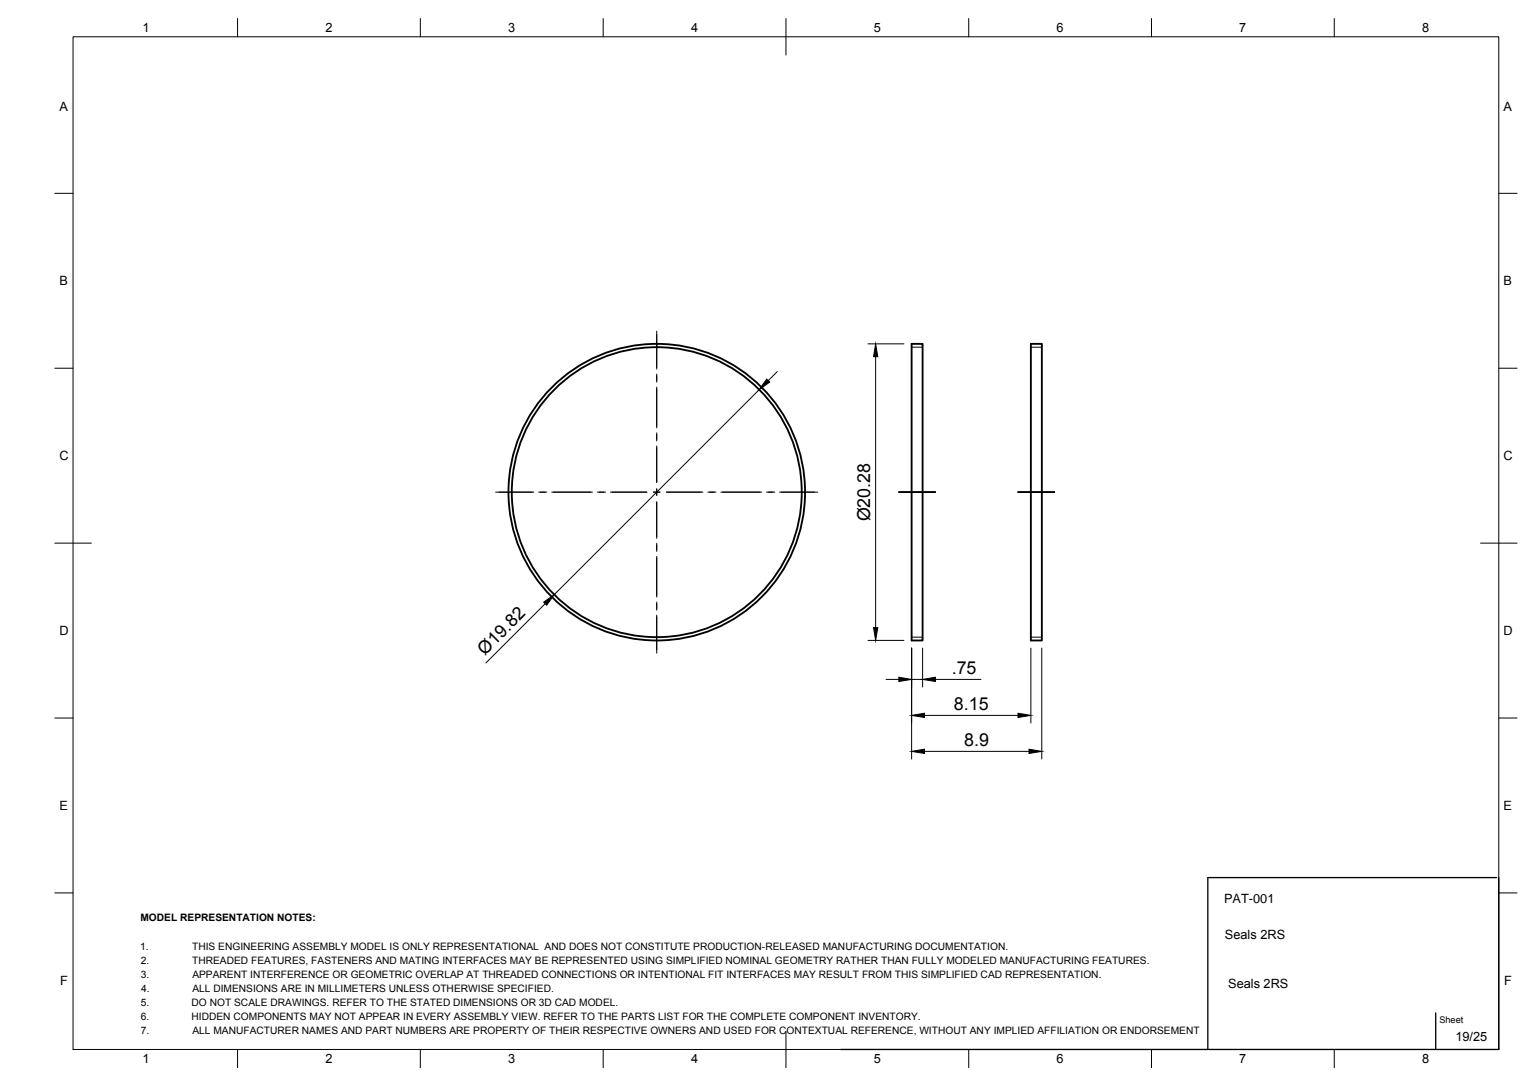
ISO-10303-21;
HEADER;
/* Generated by software containing ST-Developer
 * from STEP Tools, Inc. (www.steptools.com) 
 */

FILE_DESCRIPTION(
/* description */ ('PAT-001'),
/* implementation_level */ '2;1');

FILE_NAME(
/* name */ 'Seals 2RS.step',
/* time_stamp */ '2026-10-29T17:07:15-07:00',
/* author */ (''),
/* organization */ (''),
/* preprocessor_version */ 'ST-DEVELOPER v20.2',
/* originating_system */ 'Autodesk Translation Framework v15.17.0.0',
/* authorisation */ '');

FILE_SCHEMA (('AUTOMOTIVE_DESIGN { 1 0 10303 214 3 1 1 }'));
ENDSEC;

DATA;
#10=MECHANICAL_DESIGN_GEOMETRIC_PRESENTATION_REPRESENTATION('',(#389,#390),#9622);
#332=SHAPE_REPRESENTATION_RELATIONSHIP('SRR','None',#9756,#357);
#357=ADVANCED_BREP_SHAPE_REPRESENTATION('',(#422,#423),#9605);
#389=STYLED_ITEM('',(#9962),#422);
#390=STYLED_ITEM('',(#9962),#423);
#422=MANIFOLD_SOLID_BREP('Body1',#5214);
#423=MANIFOLD_SOLID_BREP('Body2',#5215);
#454=FACE_BOUND('',#1099,.T.);
#455=FACE_BOUND('',#1102,.T.);
#456=FACE_BOUND('',#1105,.T.);
#457=FACE_BOUND('',#1108,.T.);
#555=PLANE('',#5682);
#556=PLANE('',#5687);
#557=PLANE('',#5690);
#558=PLANE('',#5695);
#785=FACE_OUTER_BOUND('',#1098,.T.);
#786=FACE_OUTER_BOUND('',#1100,.T.);
#787=FACE_OUTER_BOUND('',#1101,.T.);
#788=FACE_OUTER_BOUND('',#1103,.T.);
#789=FACE_OUTER_BOUND('',#1104,.T.);
#790=FACE_OUTER_BOUND('',#1106,.T.);
#791=FACE_OUTER_BOUND('',#1107,.T.);
#792=FACE_OUTER_BOUND('',#1109,.T.);
#1098=EDGE_LOOP('',(#3783));
#1099=EDGE_LOOP('',(#3784));
#1100=EDGE_LOOP('',(#3785,#3786,#3787,#3788));
#1101=EDGE_LOOP('',(#3789));
#1102=EDGE_LOOP('',(#3790));
#1103=EDGE_LOOP('',(#3791,#3792,#3793,#3794));
#1104=EDGE_LOOP('',(#3795));
#1105=EDGE_LOOP('',(#3796));
#1106=EDGE_LOOP('',(#3797,#3798,#3799,#3800));
#1107=EDGE_LOOP('',(#3801));
#1108=EDGE_LOOP('',(#3802));
#1109=EDGE_LOOP('',(#3803,#3804,#3805,#3806));
#1423=LINE('',#8368,#1828);
#1424=LINE('',#8373,#1829);
#1425=LINE('',#8382,#1830);
#1426=LINE('',#8387,#1831);
#1828=VECTOR('',#6488,1.013815);
#1829=VECTOR('',#6495,0.991185);
#1830=VECTOR('',#6506,1.013815);
#1831=VECTOR('',#6513,0.991185);
#2298=CIRCLE('',#5683,1.013815);
#2299=CIRCLE('',#5684,0.991185);
#2300=CIRCLE('',#5686,1.013815);
#2301=CIRCLE('',#5688,0.991185);
#2302=CIRCLE('',#5691,1.013815);
#2303=CIRCLE('',#5692,0.991185);
#2304=CIRCLE('',#5694,1.013815);
#2305=CIRCLE('',#5696,0.991185);
#2518=VERTEX_POINT('',#8361);
#2519=VERTEX_POINT('',#8363);
#2520=VERTEX_POINT('',#8366);
#2521=VERTEX_POINT('',#8370);
#2522=VERTEX_POINT('',#8375);
#2523=VERTEX_POINT('',#8377);
#2524=VERTEX_POINT('',#8380);
#2525=VERTEX_POINT('',#8384);
#2995=EDGE_CURVE('',#2518,#2518,#2298,.T.);
#2996=EDGE_CURVE('',#2519,#2519,#2299,.T.);
#2997=EDGE_CURVE('',#2520,#2520,#2300,.T.);
#2998=EDGE_CURVE('',#2520,#2518,#1423,.T.);
#2999=EDGE_CURVE('',#2521,#2521,#2301,.T.);
#3000=EDGE_CURVE('',#2521,#2519,#1424,.T.);
#3001=EDGE_CURVE('',#2522,#2522,#2302,.T.);
#3002=EDGE_CURVE('',#2523,#2523,#2303,.T.);
#3003=EDGE_CURVE('',#2524,#2524,#2304,.T.);
#3004=EDGE_CURVE('',#2524,#2522,#1425,.T.);
#3005=EDGE_CURVE('',#2525,#2525,#2305,.T.);
#3006=EDGE_CURVE('',#2525,#2523,#1426,.T.);
#3783=ORIENTED_EDGE('',*,*,#2995,.F.);
#3784=ORIENTED_EDGE('',*,*,#2996,.T.);
#3785=ORIENTED_EDGE('',*,*,#2997,.F.);
#3786=ORIENTED_EDGE('',*,*,#2998,.T.);
#3787=ORIENTED_EDGE('',*,*,#2995,.T.);
#3788=ORIENTED_EDGE('',*,*,#2998,.F.);
#3789=ORIENTED_EDGE('',*,*,#2997,.T.);
#3790=ORIENTED_EDGE('',*,*,#2999,.F.);
#3791=ORIENTED_EDGE('',*,*,#2999,.T.);
#3792=ORIENTED_EDGE('',*,*,#3000,.T.);
#3793=ORIENTED_EDGE('',*,*,#2996,.F.);
#3794=ORIENTED_EDGE('',*,*,#3000,.F.);
#3795=ORIENTED_EDGE('',*,*,#3001,.F.);
#3796=ORIENTED_EDGE('',*,*,#3002,.T.);
#3797=ORIENTED_EDGE('',*,*,#3003,.F.);
#3798=ORIENTED_EDGE('',*,*,#3004,.T.);
#3799=ORIENTED_EDGE('',*,*,#3001,.T.);
#3800=ORIENTED_EDGE('',*,*,#3004,.F.);
#3801=ORIENTED_EDGE('',*,*,#3003,.T.);
#3802=ORIENTED_EDGE('',*,*,#3005,.F.);
#3803=ORIENTED_EDGE('',*,*,#3005,.T.);
#3804=ORIENTED_EDGE('',*,*,#3006,.T.);
#3805=ORIENTED_EDGE('',*,*,#3002,.F.);
#3806=ORIENTED_EDGE('',*,*,#3006,.F.);
#4848=CYLINDRICAL_SURFACE('',#5685,1.013815);
#4849=CYLINDRICAL_SURFACE('',#5689,0.991185);
#4850=CYLINDRICAL_SURFACE('',#5693,1.013815);
#4851=CYLINDRICAL_SURFACE('',#5697,0.991185);
#4972=ADVANCED_FACE('',(#785,#454),#555,.T.);
#4973=ADVANCED_FACE('',(#786),#4848,.T.);
#4974=ADVANCED_FACE('',(#787,#455),#556,.T.);
#4975=ADVANCED_FACE('',(#788),#4849,.F.);
#4976=ADVANCED_FACE('',(#789,#456),#557,.T.);
#4977=ADVANCED_FACE('',(#790),#4850,.T.);
#4978=ADVANCED_FACE('',(#791,#457),#558,.T.);
#4979=ADVANCED_FACE('',(#792),#4851,.F.);
#5214=CLOSED_SHELL('',(#4972,#4973,#4974,#4975));
#5215=CLOSED_SHELL('',(#4976,#4977,#4978,#4979));
#5681=AXIS2_PLACEMENT_3D('',#8359,#6476,#6477);
#5682=AXIS2_PLACEMENT_3D('',#8360,#6478,#6479);
#5683=AXIS2_PLACEMENT_3D('',#8362,#6480,#6481);
#5684=AXIS2_PLACEMENT_3D('',#8364,#6482,#6483);
#5685=AXIS2_PLACEMENT_3D('',#8365,#6484,#6485);
#5686=AXIS2_PLACEMENT_3D('',#8367,#6486,#6487);
#5687=AXIS2_PLACEMENT_3D('',#8369,#6489,#6490);
#5688=AXIS2_PLACEMENT_3D('',#8371,#6491,#6492);
#5689=AXIS2_PLACEMENT_3D('',#8372,#6493,#6494);
#5690=AXIS2_PLACEMENT_3D('',#8374,#6496,#6497);
#5691=AXIS2_PLACEMENT_3D('',#8376,#6498,#6499);
#5692=AXIS2_PLACEMENT_3D('',#8378,#6500,#6501);
#5693=AXIS2_PLACEMENT_3D('',#8379,#6502,#6503);
#5694=AXIS2_PLACEMENT_3D('',#8381,#6504,#6505);
#5695=AXIS2_PLACEMENT_3D('',#8383,#6507,#6508);
#5696=AXIS2_PLACEMENT_3D('',#8385,#6509,#6510);
#5697=AXIS2_PLACEMENT_3D('',#8386,#6511,#6512);
#6476=DIRECTION('axis',(0.,0.,1.));
#6477=DIRECTION('refdir',(1.,0.,0.));
#6478=DIRECTION('center_axis',(0.,1.,0.));
#6479=DIRECTION('ref_axis',(0.,0.,1.));
#6480=DIRECTION('center_axis',(0.,-1.,0.));
#6481=DIRECTION('ref_axis',(1.,0.,0.));
#6482=DIRECTION('center_axis',(0.,-1.,0.));
#6483=DIRECTION('ref_axis',(1.,0.,0.));
#6484=DIRECTION('center_axis',(0.,-1.,0.));
#6485=DIRECTION('ref_axis',(1.,0.,0.));
#6486=DIRECTION('center_axis',(0.,-1.,0.));
#6487=DIRECTION('ref_axis',(1.,0.,0.));
#6488=DIRECTION('',(0.,1.,0.));
#6489=DIRECTION('center_axis',(0.,-1.,0.));
#6490=DIRECTION('ref_axis',(0.,0.,-1.));
#6491=DIRECTION('center_axis',(0.,-1.,0.));
#6492=DIRECTION('ref_axis',(1.,0.,0.));
#6493=DIRECTION('center_axis',(0.,-1.,0.));
#6494=DIRECTION('ref_axis',(1.,0.,0.));
#6495=DIRECTION('',(0.,1.,0.));
#6496=DIRECTION('center_axis',(0.,1.,0.));
#6497=DIRECTION('ref_axis',(0.,0.,1.));
#6498=DIRECTION('center_axis',(0.,-1.,0.));
#6499=DIRECTION('ref_axis',(1.,0.,0.));
#6500=DIRECTION('center_axis',(0.,-1.,0.));
#6501=DIRECTION('ref_axis',(1.,0.,0.));
#6502=DIRECTION('center_axis',(0.,-1.,0.));
#6503=DIRECTION('ref_axis',(1.,0.,0.));
#6504=DIRECTION('center_axis',(0.,-1.,0.));
#6505=DIRECTION('ref_axis',(1.,0.,0.));
#6506=DIRECTION('',(0.,1.,0.));
#6507=DIRECTION('center_axis',(0.,-1.,0.));
#6508=DIRECTION('ref_axis',(0.,0.,-1.));
#6509=DIRECTION('center_axis',(0.,-1.,0.));
#6510=DIRECTION('ref_axis',(1.,0.,0.));
#6511=DIRECTION('center_axis',(0.,-1.,0.));
#6512=DIRECTION('ref_axis',(1.,0.,0.));
#6513=DIRECTION('',(0.,1.,0.));
#8359=CARTESIAN_POINT('',(0.,0.,0.));
#8360=CARTESIAN_POINT('Origin',(1.013815,0.445,0.));
#8361=CARTESIAN_POINT('',(-1.013815,0.445,-1.24156529467757E-16));
#8362=CARTESIAN_POINT('Origin',(0.,0.445,0.));
#8363=CARTESIAN_POINT('',(-0.991185,0.445,-1.21385153761287E-16));
#8364=CARTESIAN_POINT('Origin',(0.,0.445,0.));
#8365=CARTESIAN_POINT('Origin',(0.,0.4075,0.));
#8366=CARTESIAN_POINT('',(-1.013815,0.37,-1.24156529467757E-16));
#8367=CARTESIAN_POINT('Origin',(0.,0.37,0.));
#8368=CARTESIAN_POINT('',(-1.013815,0.4075,-1.24156529467757E-16));
#8369=CARTESIAN_POINT('Origin',(0.991185,0.37,0.));
#8370=CARTESIAN_POINT('',(-0.991185,0.37,-1.21385153761287E-16));
#8371=CARTESIAN_POINT('Origin',(0.,0.37,0.));
#8372=CARTESIAN_POINT('Origin',(0.,0.4075,0.));
#8373=CARTESIAN_POINT('',(-0.991185,0.4075,-1.21385153761287E-16));
#8374=CARTESIAN_POINT('Origin',(1.013815,-0.37,0.));
#8375=CARTESIAN_POINT('',(-1.013815,-0.37,-1.24156529467757E-16));
#8376=CARTESIAN_POINT('Origin',(0.,-0.37,0.));
#8377=CARTESIAN_POINT('',(-0.991185,-0.37,-1.21385153761287E-16));
#8378=CARTESIAN_POINT('Origin',(0.,-0.37,0.));
#8379=CARTESIAN_POINT('Origin',(0.,-0.4075,0.));
#8380=CARTESIAN_POINT('',(-1.013815,-0.445,-1.24156529467757E-16));
#8381=CARTESIAN_POINT('Origin',(0.,-0.445,0.));
#8382=CARTESIAN_POINT('',(-1.013815,-0.4075,-1.24156529467757E-16));
#8383=CARTESIAN_POINT('Origin',(0.991185,-0.445,0.));
#8384=CARTESIAN_POINT('',(-0.991185,-0.445,-1.21385153761287E-16));
#8385=CARTESIAN_POINT('Origin',(0.,-0.445,0.));
#8386=CARTESIAN_POINT('Origin',(0.,-0.4075,0.));
#8387=CARTESIAN_POINT('',(-0.991185,-0.4075,-1.21385153761287E-16));
#9575=UNCERTAINTY_MEASURE_WITH_UNIT(LENGTH_MEASURE(0.001),#9623,
'DISTANCE_ACCURACY_VALUE',
'Maximum model space distance between geometric entities at asserted c
onnectivities');
#9592=UNCERTAINTY_MEASURE_WITH_UNIT(LENGTH_MEASURE(0.001),#9623,
'DISTANCE_ACCURACY_VALUE',
'Maximum model space distance between geometric entities at asserted c
onnectivities');
#9605=(
GEOMETRIC_REPRESENTATION_CONTEXT(3)
GLOBAL_UNCERTAINTY_ASSIGNED_CONTEXT((#9575))
GLOBAL_UNIT_ASSIGNED_CONTEXT((#9623,#9625,#9626))
REPRESENTATION_CONTEXT('','3D')
);
#9622=(
GEOMETRIC_REPRESENTATION_CONTEXT(3)
GLOBAL_UNCERTAINTY_ASSIGNED_CONTEXT((#9592))
GLOBAL_UNIT_ASSIGNED_CONTEXT((#9623,#9625,#9626))
REPRESENTATION_CONTEXT('','3D')
);
#9623=(
LENGTH_UNIT()
NAMED_UNIT(*)
SI_UNIT(.CENTI.,.METRE.)
);
#9625=(
NAMED_UNIT(*)
PLANE_ANGLE_UNIT()
SI_UNIT($,.RADIAN.)
);
#9626=(
NAMED_UNIT(*)
SI_UNIT($,.STERADIAN.)
SOLID_ANGLE_UNIT()
);
#9639=SHAPE_DEFINITION_REPRESENTATION(#9668,#9756);
#9668=PRODUCT_DEFINITION_SHAPE('',$,#9786);
#9756=SHAPE_REPRESENTATION('',(#5681),#9605);
#9773=PRODUCT_DEFINITION_CONTEXT('part definition',#9862,'design');
#9786=PRODUCT_DEFINITION('Seals 2RS','Seals 2RS',#9815,#9773);
#9815=PRODUCT_DEFINITION_FORMATION('',$,#9876);
#9862=APPLICATION_CONTEXT(
'Core Data for Automotive Mechanical Design Process');
#9863=PRODUCT_CONTEXT('part definition',#9862,'mechanical');
#9876=PRODUCT('Seals 2RS','Seals 2RS','Seals 2RS',(#9863));
#9956=COLOUR_RGB('Grey',0.48,0.52,0.57);
#9957=FILL_AREA_STYLE_COLOUR('',#9956);
#9958=FILL_AREA_STYLE('',(#9957));
#9959=SURFACE_STYLE_FILL_AREA(#9958);
#9960=SURFACE_SIDE_STYLE('',(#9959));
#9961=SURFACE_STYLE_USAGE(.BOTH.,#9960);
#9962=PRESENTATION_STYLE_ASSIGNMENT((#9961));
ENDSEC;
END-ISO-10303-21;
